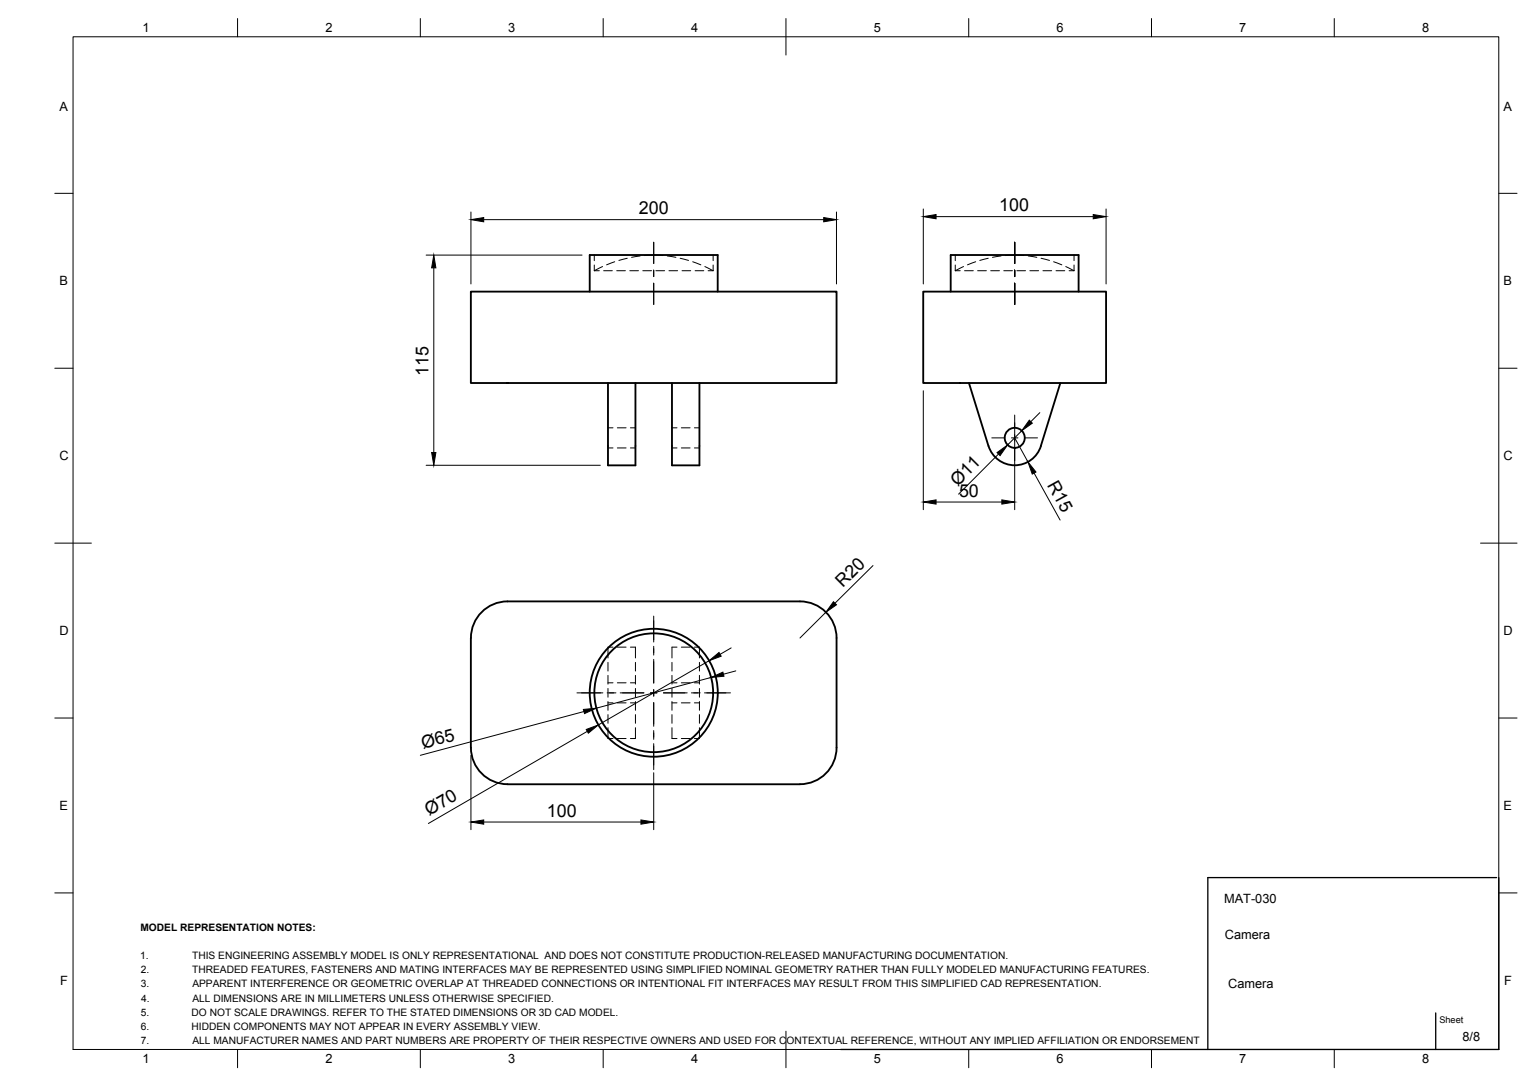
ISO-10303-21;
HEADER;
/* Generated by software containing ST-Developer
 * from STEP Tools, Inc. (www.steptools.com) 
 */

FILE_DESCRIPTION(
/* description */ ('STEP AP214'),
/* implementation_level */ '2;1');

FILE_NAME(
/* name */ 'Camera.step',
/* time_stamp */ '2026-11-14T06:43:04-08:00',
/* author */ (''),
/* organization */ (''),
/* preprocessor_version */ 'ST-DEVELOPER v20.2',
/* originating_system */ 'Autodesk Translation Framework v15.17.0.0',
/* authorisation */ '');

FILE_SCHEMA (('AUTOMOTIVE_DESIGN { 1 0 10303 214 3 1 1 }'));
ENDSEC;

DATA;
#10=MECHANICAL_DESIGN_GEOMETRIC_PRESENTATION_REPRESENTATION('',(#201),#5658);
#165=(
BOUNDED_SURFACE()
B_SPLINE_SURFACE(2,2,((#4850,#4851,#4852,#4853,#4854,#4855,#4856,#4857,
#4858),(#4859,#4860,#4861,#4862,#4863,#4864,#4865,#4866,#4867),(#4868,#4869,
#4870,#4871,#4872,#4873,#4874,#4875,#4876)),.UNSPECIFIED.,.F.,.T.,.F.)
B_SPLINE_SURFACE_WITH_KNOTS((3,3),(3,2,2,2,3),(-1.55552293509789,-1.0706447979528),
(-3.14159265358979,-1.5707963267949,0.,1.5707963267949,3.14159265358979),
 .UNSPECIFIED.)
GEOMETRIC_REPRESENTATION_ITEM()
RATIONAL_B_SPLINE_SURFACE(((1.,0.707106781186548,1.,0.707106781186548,1.,
0.707106781186548,1.,0.707106781186548,1.),(0.970755313150814,0.686427664801811,
0.970755313150814,0.686427664801811,0.970755313150814,0.686427664801811,
0.970755313150814,0.686427664801811,0.970755313150814),(1.,0.707106781186548,
1.,0.707106781186548,1.,0.707106781186548,1.,0.707106781186548,1.)))
REPRESENTATION_ITEM('')
SURFACE()
);
#179=SHAPE_REPRESENTATION_RELATIONSHIP('SRR','None',#5709,#190);
#190=ADVANCED_BREP_SHAPE_REPRESENTATION('',(#212),#5650);
#201=STYLED_ITEM('',(#5772),#212);
#212=MANIFOLD_SOLID_BREP('Body1',#3063);
#242=CYLINDRICAL_SURFACE('',#3279,5.5);
#243=CYLINDRICAL_SURFACE('',#3282,5.5);
#244=CYLINDRICAL_SURFACE('',#3285,35.);
#245=CYLINDRICAL_SURFACE('',#3290,32.5);
#246=CYLINDRICAL_SURFACE('',#3292,15.);
#247=CYLINDRICAL_SURFACE('',#3297,20.);
#248=CYLINDRICAL_SURFACE('',#3301,20.);
#249=CYLINDRICAL_SURFACE('',#3305,20.);
#250=CYLINDRICAL_SURFACE('',#3309,20.);
#251=CYLINDRICAL_SURFACE('',#3316,15.);
#299=FACE_BOUND('',#603,.T.);
#300=FACE_BOUND('',#604,.T.);
#301=FACE_BOUND('',#606,.T.);
#302=FACE_BOUND('',#608,.T.);
#303=FACE_BOUND('',#613,.T.);
#304=FACE_BOUND('',#615,.T.);
#305=FACE_BOUND('',#617,.T.);
#306=FACE_BOUND('',#619,.T.);
#376=FACE_OUTER_BOUND('',#586,.T.);
#377=FACE_OUTER_BOUND('',#587,.T.);
#378=FACE_OUTER_BOUND('',#588,.T.);
#379=FACE_OUTER_BOUND('',#589,.T.);
#380=FACE_OUTER_BOUND('',#590,.T.);
#381=FACE_OUTER_BOUND('',#591,.T.);
#382=FACE_OUTER_BOUND('',#592,.T.);
#383=FACE_OUTER_BOUND('',#593,.T.);
#384=FACE_OUTER_BOUND('',#594,.T.);
#385=FACE_OUTER_BOUND('',#595,.T.);
#386=FACE_OUTER_BOUND('',#596,.T.);
#387=FACE_OUTER_BOUND('',#597,.T.);
#388=FACE_OUTER_BOUND('',#598,.T.);
#389=FACE_OUTER_BOUND('',#599,.T.);
#390=FACE_OUTER_BOUND('',#600,.T.);
#391=FACE_OUTER_BOUND('',#601,.T.);
#392=FACE_OUTER_BOUND('',#602,.T.);
#393=FACE_OUTER_BOUND('',#605,.T.);
#394=FACE_OUTER_BOUND('',#607,.T.);
#395=FACE_OUTER_BOUND('',#609,.T.);
#396=FACE_OUTER_BOUND('',#610,.T.);
#397=FACE_OUTER_BOUND('',#611,.T.);
#398=FACE_OUTER_BOUND('',#612,.T.);
#399=FACE_OUTER_BOUND('',#614,.T.);
#400=FACE_OUTER_BOUND('',#616,.T.);
#401=FACE_OUTER_BOUND('',#618,.T.);
#586=EDGE_LOOP('',(#2158,#2159,#2160,#2161));
#587=EDGE_LOOP('',(#2162,#2163,#2164,#2165));
#588=EDGE_LOOP('',(#2166,#2167,#2168,#2169));
#589=EDGE_LOOP('',(#2170,#2171,#2172));
#590=EDGE_LOOP('',(#2173,#2174,#2175,#2176));
#591=EDGE_LOOP('',(#2177,#2178,#2179,#2180));
#592=EDGE_LOOP('',(#2181,#2182,#2183,#2184));
#593=EDGE_LOOP('',(#2185,#2186,#2187,#2188));
#594=EDGE_LOOP('',(#2189,#2190,#2191,#2192));
#595=EDGE_LOOP('',(#2193,#2194,#2195,#2196));
#596=EDGE_LOOP('',(#2197,#2198,#2199,#2200));
#597=EDGE_LOOP('',(#2201,#2202,#2203,#2204));
#598=EDGE_LOOP('',(#2205,#2206,#2207,#2208));
#599=EDGE_LOOP('',(#2209,#2210,#2211,#2212));
#600=EDGE_LOOP('',(#2213,#2214,#2215,#2216));
#601=EDGE_LOOP('',(#2217,#2218,#2219,#2220));
#602=EDGE_LOOP('',(#2221,#2222,#2223,#2224,#2225,#2226,#2227,#2228));
#603=EDGE_LOOP('',(#2229,#2230,#2231,#2232));
#604=EDGE_LOOP('',(#2233,#2234,#2235,#2236));
#605=EDGE_LOOP('',(#2237,#2238,#2239,#2240,#2241,#2242,#2243,#2244));
#606=EDGE_LOOP('',(#2245));
#607=EDGE_LOOP('',(#2246));
#608=EDGE_LOOP('',(#2247));
#609=EDGE_LOOP('',(#2248,#2249,#2250,#2251));
#610=EDGE_LOOP('',(#2252,#2253,#2254,#2255));
#611=EDGE_LOOP('',(#2256,#2257,#2258,#2259));
#612=EDGE_LOOP('',(#2260,#2261,#2262,#2263));
#613=EDGE_LOOP('',(#2264));
#614=EDGE_LOOP('',(#2265,#2266,#2267,#2268));
#615=EDGE_LOOP('',(#2269));
#616=EDGE_LOOP('',(#2270,#2271,#2272,#2273));
#617=EDGE_LOOP('',(#2274));
#618=EDGE_LOOP('',(#2275,#2276,#2277,#2278));
#619=EDGE_LOOP('',(#2279));
#810=LINE('',#4836,#1006);
#811=LINE('',#4842,#1007);
#812=LINE('',#4848,#1008);
#813=LINE('',#4884,#1009);
#814=LINE('',#4890,#1010);
#815=LINE('',#4893,#1011);
#816=LINE('',#4896,#1012);
#817=LINE('',#4898,#1013);
#818=LINE('',#4899,#1014);
#819=LINE('',#4902,#1015);
#820=LINE('',#4904,#1016);
#821=LINE('',#4905,#1017);
#822=LINE('',#4911,#1018);
#823=LINE('',#4914,#1019);
#824=LINE('',#4917,#1020);
#825=LINE('',#4919,#1021);
#826=LINE('',#4920,#1022);
#827=LINE('',#4925,#1023);
#828=LINE('',#4929,#1024);
#829=LINE('',#4931,#1025);
#830=LINE('',#4932,#1026);
#831=LINE('',#4937,#1027);
#832=LINE('',#4941,#1028);
#833=LINE('',#4943,#1029);
#834=LINE('',#4944,#1030);
#835=LINE('',#4949,#1031);
#836=LINE('',#4952,#1032);
#837=LINE('',#4953,#1033);
#838=LINE('',#4957,#1034);
#839=LINE('',#4959,#1035);
#840=LINE('',#4961,#1036);
#841=LINE('',#4962,#1037);
#842=LINE('',#4963,#1038);
#843=LINE('',#4964,#1039);
#844=LINE('',#4970,#1040);
#845=LINE('',#4974,#1041);
#846=LINE('',#4977,#1042);
#847=LINE('',#4978,#1043);
#848=LINE('',#4980,#1044);
#849=LINE('',#4981,#1045);
#1006=VECTOR('',#3778,5.5);
#1007=VECTOR('',#3785,5.5);
#1008=VECTOR('',#3792,35.);
#1009=VECTOR('',#3803,32.5);
#1010=VECTOR('',#3808,1000.);
#1011=VECTOR('',#3811,1000.);
#1012=VECTOR('',#3814,1000.);
#1013=VECTOR('',#3815,1000.);
#1014=VECTOR('',#3816,1000.);
#1015=VECTOR('',#3819,1000.);
#1016=VECTOR('',#3820,1000.);
#1017=VECTOR('',#3821,1000.);
#1018=VECTOR('',#3826,1000.);
#1019=VECTOR('',#3829,1000.);
#1020=VECTOR('',#3832,1000.);
#1021=VECTOR('',#3833,1000.);
#1022=VECTOR('',#3834,1000.);
#1023=VECTOR('',#3839,1000.);
#1024=VECTOR('',#3844,1000.);
#1025=VECTOR('',#3845,1000.);
#1026=VECTOR('',#3846,1000.);
#1027=VECTOR('',#3851,1000.);
#1028=VECTOR('',#3856,1000.);
#1029=VECTOR('',#3857,1000.);
#1030=VECTOR('',#3858,1000.);
#1031=VECTOR('',#3863,1000.);
#1032=VECTOR('',#3868,1000.);
#1033=VECTOR('',#3869,1000.);
#1034=VECTOR('',#3872,1000.);
#1035=VECTOR('',#3873,1000.);
#1036=VECTOR('',#3874,1000.);
#1037=VECTOR('',#3875,1000.);
#1038=VECTOR('',#3876,1000.);
#1039=VECTOR('',#3877,1000.);
#1040=VECTOR('',#3884,1000.);
#1041=VECTOR('',#3887,1000.);
#1042=VECTOR('',#3892,1000.);
#1043=VECTOR('',#3893,1000.);
#1044=VECTOR('',#3896,1000.);
#1045=VECTOR('',#3897,1000.);
#1201=CIRCLE('',#3280,5.5);
#1202=CIRCLE('',#3281,5.5);
#1203=CIRCLE('',#3283,5.5);
#1204=CIRCLE('',#3284,5.5);
#1205=CIRCLE('',#3286,35.);
#1206=CIRCLE('',#3287,35.);
#1207=CIRCLE('',#3288,32.5);
#1208=CIRCLE('',#3289,70.);
#1209=CIRCLE('',#3291,32.5);
#1210=CIRCLE('',#3293,15.);
#1211=CIRCLE('',#3294,15.);
#1212=CIRCLE('',#3298,20.);
#1213=CIRCLE('',#3299,20.);
#1214=CIRCLE('',#3302,20.);
#1215=CIRCLE('',#3303,20.);
#1216=CIRCLE('',#3306,20.);
#1217=CIRCLE('',#3307,20.);
#1218=CIRCLE('',#3310,20.);
#1219=CIRCLE('',#3311,20.);
#1220=CIRCLE('',#3317,15.);
#1221=CIRCLE('',#3318,15.);
#1374=VERTEX_POINT('',#4833);
#1375=VERTEX_POINT('',#4835);
#1376=VERTEX_POINT('',#4839);
#1377=VERTEX_POINT('',#4841);
#1378=VERTEX_POINT('',#4845);
#1379=VERTEX_POINT('',#4847);
#1380=VERTEX_POINT('',#4877);
#1381=VERTEX_POINT('',#4879);
#1382=VERTEX_POINT('',#4882);
#1383=VERTEX_POINT('',#4886);
#1384=VERTEX_POINT('',#4887);
#1385=VERTEX_POINT('',#4889);
#1386=VERTEX_POINT('',#4891);
#1387=VERTEX_POINT('',#4895);
#1388=VERTEX_POINT('',#4897);
#1389=VERTEX_POINT('',#4901);
#1390=VERTEX_POINT('',#4903);
#1391=VERTEX_POINT('',#4907);
#1392=VERTEX_POINT('',#4908);
#1393=VERTEX_POINT('',#4910);
#1394=VERTEX_POINT('',#4912);
#1395=VERTEX_POINT('',#4916);
#1396=VERTEX_POINT('',#4918);
#1397=VERTEX_POINT('',#4922);
#1398=VERTEX_POINT('',#4924);
#1399=VERTEX_POINT('',#4928);
#1400=VERTEX_POINT('',#4930);
#1401=VERTEX_POINT('',#4934);
#1402=VERTEX_POINT('',#4936);
#1403=VERTEX_POINT('',#4940);
#1404=VERTEX_POINT('',#4942);
#1405=VERTEX_POINT('',#4946);
#1406=VERTEX_POINT('',#4948);
#1407=VERTEX_POINT('',#4955);
#1408=VERTEX_POINT('',#4956);
#1409=VERTEX_POINT('',#4958);
#1410=VERTEX_POINT('',#4960);
#1411=VERTEX_POINT('',#4968);
#1412=VERTEX_POINT('',#4969);
#1413=VERTEX_POINT('',#4971);
#1414=VERTEX_POINT('',#4973);
#1662=EDGE_CURVE('',#1374,#1374,#1201,.T.);
#1663=EDGE_CURVE('',#1374,#1375,#810,.T.);
#1664=EDGE_CURVE('',#1375,#1375,#1202,.T.);
#1665=EDGE_CURVE('',#1376,#1376,#1203,.T.);
#1666=EDGE_CURVE('',#1376,#1377,#811,.T.);
#1667=EDGE_CURVE('',#1377,#1377,#1204,.T.);
#1668=EDGE_CURVE('',#1378,#1378,#1205,.T.);
#1669=EDGE_CURVE('',#1378,#1379,#812,.T.);
#1670=EDGE_CURVE('',#1379,#1379,#1206,.T.);
#1671=EDGE_CURVE('',#1380,#1380,#1207,.T.);
#1672=EDGE_CURVE('',#1380,#1381,#1208,.T.);
#1673=EDGE_CURVE('',#1382,#1382,#1209,.T.);
#1674=EDGE_CURVE('',#1382,#1380,#813,.T.);
#1675=EDGE_CURVE('',#1383,#1384,#1210,.T.);
#1676=EDGE_CURVE('',#1383,#1385,#814,.T.);
#1677=EDGE_CURVE('',#1385,#1386,#1211,.T.);
#1678=EDGE_CURVE('',#1384,#1386,#815,.T.);
#1679=EDGE_CURVE('',#1384,#1387,#816,.T.);
#1680=EDGE_CURVE('',#1386,#1388,#817,.T.);
#1681=EDGE_CURVE('',#1387,#1388,#818,.T.);
#1682=EDGE_CURVE('',#1389,#1383,#819,.T.);
#1683=EDGE_CURVE('',#1389,#1390,#820,.T.);
#1684=EDGE_CURVE('',#1390,#1385,#821,.T.);
#1685=EDGE_CURVE('',#1391,#1392,#1212,.T.);
#1686=EDGE_CURVE('',#1393,#1391,#822,.T.);
#1687=EDGE_CURVE('',#1393,#1394,#1213,.T.);
#1688=EDGE_CURVE('',#1394,#1392,#823,.T.);
#1689=EDGE_CURVE('',#1395,#1391,#824,.T.);
#1690=EDGE_CURVE('',#1396,#1395,#825,.T.);
#1691=EDGE_CURVE('',#1396,#1393,#826,.T.);
#1692=EDGE_CURVE('',#1397,#1395,#1214,.T.);
#1693=EDGE_CURVE('',#1398,#1397,#827,.T.);
#1694=EDGE_CURVE('',#1398,#1396,#1215,.T.);
#1695=EDGE_CURVE('',#1399,#1397,#828,.T.);
#1696=EDGE_CURVE('',#1400,#1399,#829,.T.);
#1697=EDGE_CURVE('',#1400,#1398,#830,.T.);
#1698=EDGE_CURVE('',#1401,#1399,#1216,.T.);
#1699=EDGE_CURVE('',#1402,#1401,#831,.T.);
#1700=EDGE_CURVE('',#1402,#1400,#1217,.T.);
#1701=EDGE_CURVE('',#1403,#1401,#832,.T.);
#1702=EDGE_CURVE('',#1404,#1403,#833,.T.);
#1703=EDGE_CURVE('',#1404,#1402,#834,.T.);
#1704=EDGE_CURVE('',#1405,#1403,#1218,.T.);
#1705=EDGE_CURVE('',#1406,#1405,#835,.T.);
#1706=EDGE_CURVE('',#1406,#1404,#1219,.T.);
#1707=EDGE_CURVE('',#1392,#1405,#836,.T.);
#1708=EDGE_CURVE('',#1394,#1406,#837,.T.);
#1709=EDGE_CURVE('',#1407,#1408,#838,.T.);
#1710=EDGE_CURVE('',#1408,#1409,#839,.T.);
#1711=EDGE_CURVE('',#1410,#1409,#840,.T.);
#1712=EDGE_CURVE('',#1407,#1410,#841,.T.);
#1713=EDGE_CURVE('',#1387,#1389,#842,.T.);
#1714=EDGE_CURVE('',#1388,#1390,#843,.T.);
#1715=EDGE_CURVE('',#1411,#1412,#844,.T.);
#1716=EDGE_CURVE('',#1412,#1413,#1220,.T.);
#1717=EDGE_CURVE('',#1414,#1413,#845,.T.);
#1718=EDGE_CURVE('',#1411,#1414,#1221,.T.);
#1719=EDGE_CURVE('',#1413,#1408,#846,.T.);
#1720=EDGE_CURVE('',#1414,#1407,#847,.T.);
#1721=EDGE_CURVE('',#1409,#1412,#848,.T.);
#1722=EDGE_CURVE('',#1410,#1411,#849,.T.);
#2158=ORIENTED_EDGE('',*,*,#1662,.F.);
#2159=ORIENTED_EDGE('',*,*,#1663,.T.);
#2160=ORIENTED_EDGE('',*,*,#1664,.T.);
#2161=ORIENTED_EDGE('',*,*,#1663,.F.);
#2162=ORIENTED_EDGE('',*,*,#1665,.F.);
#2163=ORIENTED_EDGE('',*,*,#1666,.T.);
#2164=ORIENTED_EDGE('',*,*,#1667,.T.);
#2165=ORIENTED_EDGE('',*,*,#1666,.F.);
#2166=ORIENTED_EDGE('',*,*,#1668,.F.);
#2167=ORIENTED_EDGE('',*,*,#1669,.T.);
#2168=ORIENTED_EDGE('',*,*,#1670,.T.);
#2169=ORIENTED_EDGE('',*,*,#1669,.F.);
#2170=ORIENTED_EDGE('',*,*,#1671,.F.);
#2171=ORIENTED_EDGE('',*,*,#1672,.T.);
#2172=ORIENTED_EDGE('',*,*,#1672,.F.);
#2173=ORIENTED_EDGE('',*,*,#1673,.F.);
#2174=ORIENTED_EDGE('',*,*,#1674,.T.);
#2175=ORIENTED_EDGE('',*,*,#1671,.T.);
#2176=ORIENTED_EDGE('',*,*,#1674,.F.);
#2177=ORIENTED_EDGE('',*,*,#1675,.F.);
#2178=ORIENTED_EDGE('',*,*,#1676,.T.);
#2179=ORIENTED_EDGE('',*,*,#1677,.T.);
#2180=ORIENTED_EDGE('',*,*,#1678,.F.);
#2181=ORIENTED_EDGE('',*,*,#1679,.F.);
#2182=ORIENTED_EDGE('',*,*,#1678,.T.);
#2183=ORIENTED_EDGE('',*,*,#1680,.T.);
#2184=ORIENTED_EDGE('',*,*,#1681,.F.);
#2185=ORIENTED_EDGE('',*,*,#1682,.F.);
#2186=ORIENTED_EDGE('',*,*,#1683,.T.);
#2187=ORIENTED_EDGE('',*,*,#1684,.T.);
#2188=ORIENTED_EDGE('',*,*,#1676,.F.);
#2189=ORIENTED_EDGE('',*,*,#1685,.F.);
#2190=ORIENTED_EDGE('',*,*,#1686,.F.);
#2191=ORIENTED_EDGE('',*,*,#1687,.T.);
#2192=ORIENTED_EDGE('',*,*,#1688,.T.);
#2193=ORIENTED_EDGE('',*,*,#1689,.F.);
#2194=ORIENTED_EDGE('',*,*,#1690,.F.);
#2195=ORIENTED_EDGE('',*,*,#1691,.T.);
#2196=ORIENTED_EDGE('',*,*,#1686,.T.);
#2197=ORIENTED_EDGE('',*,*,#1692,.F.);
#2198=ORIENTED_EDGE('',*,*,#1693,.F.);
#2199=ORIENTED_EDGE('',*,*,#1694,.T.);
#2200=ORIENTED_EDGE('',*,*,#1690,.T.);
#2201=ORIENTED_EDGE('',*,*,#1695,.F.);
#2202=ORIENTED_EDGE('',*,*,#1696,.F.);
#2203=ORIENTED_EDGE('',*,*,#1697,.T.);
#2204=ORIENTED_EDGE('',*,*,#1693,.T.);
#2205=ORIENTED_EDGE('',*,*,#1698,.F.);
#2206=ORIENTED_EDGE('',*,*,#1699,.F.);
#2207=ORIENTED_EDGE('',*,*,#1700,.T.);
#2208=ORIENTED_EDGE('',*,*,#1696,.T.);
#2209=ORIENTED_EDGE('',*,*,#1701,.F.);
#2210=ORIENTED_EDGE('',*,*,#1702,.F.);
#2211=ORIENTED_EDGE('',*,*,#1703,.T.);
#2212=ORIENTED_EDGE('',*,*,#1699,.T.);
#2213=ORIENTED_EDGE('',*,*,#1704,.F.);
#2214=ORIENTED_EDGE('',*,*,#1705,.F.);
#2215=ORIENTED_EDGE('',*,*,#1706,.T.);
#2216=ORIENTED_EDGE('',*,*,#1702,.T.);
#2217=ORIENTED_EDGE('',*,*,#1707,.F.);
#2218=ORIENTED_EDGE('',*,*,#1688,.F.);
#2219=ORIENTED_EDGE('',*,*,#1708,.T.);
#2220=ORIENTED_EDGE('',*,*,#1705,.T.);
#2221=ORIENTED_EDGE('',*,*,#1687,.F.);
#2222=ORIENTED_EDGE('',*,*,#1691,.F.);
#2223=ORIENTED_EDGE('',*,*,#1694,.F.);
#2224=ORIENTED_EDGE('',*,*,#1697,.F.);
#2225=ORIENTED_EDGE('',*,*,#1700,.F.);
#2226=ORIENTED_EDGE('',*,*,#1703,.F.);
#2227=ORIENTED_EDGE('',*,*,#1706,.F.);
#2228=ORIENTED_EDGE('',*,*,#1708,.F.);
#2229=ORIENTED_EDGE('',*,*,#1709,.T.);
#2230=ORIENTED_EDGE('',*,*,#1710,.T.);
#2231=ORIENTED_EDGE('',*,*,#1711,.F.);
#2232=ORIENTED_EDGE('',*,*,#1712,.F.);
#2233=ORIENTED_EDGE('',*,*,#1713,.F.);
#2234=ORIENTED_EDGE('',*,*,#1681,.T.);
#2235=ORIENTED_EDGE('',*,*,#1714,.T.);
#2236=ORIENTED_EDGE('',*,*,#1683,.F.);
#2237=ORIENTED_EDGE('',*,*,#1685,.T.);
#2238=ORIENTED_EDGE('',*,*,#1707,.T.);
#2239=ORIENTED_EDGE('',*,*,#1704,.T.);
#2240=ORIENTED_EDGE('',*,*,#1701,.T.);
#2241=ORIENTED_EDGE('',*,*,#1698,.T.);
#2242=ORIENTED_EDGE('',*,*,#1695,.T.);
#2243=ORIENTED_EDGE('',*,*,#1692,.T.);
#2244=ORIENTED_EDGE('',*,*,#1689,.T.);
#2245=ORIENTED_EDGE('',*,*,#1668,.T.);
#2246=ORIENTED_EDGE('',*,*,#1670,.F.);
#2247=ORIENTED_EDGE('',*,*,#1673,.T.);
#2248=ORIENTED_EDGE('',*,*,#1715,.T.);
#2249=ORIENTED_EDGE('',*,*,#1716,.T.);
#2250=ORIENTED_EDGE('',*,*,#1717,.F.);
#2251=ORIENTED_EDGE('',*,*,#1718,.F.);
#2252=ORIENTED_EDGE('',*,*,#1717,.T.);
#2253=ORIENTED_EDGE('',*,*,#1719,.T.);
#2254=ORIENTED_EDGE('',*,*,#1709,.F.);
#2255=ORIENTED_EDGE('',*,*,#1720,.F.);
#2256=ORIENTED_EDGE('',*,*,#1711,.T.);
#2257=ORIENTED_EDGE('',*,*,#1721,.T.);
#2258=ORIENTED_EDGE('',*,*,#1715,.F.);
#2259=ORIENTED_EDGE('',*,*,#1722,.F.);
#2260=ORIENTED_EDGE('',*,*,#1718,.T.);
#2261=ORIENTED_EDGE('',*,*,#1720,.T.);
#2262=ORIENTED_EDGE('',*,*,#1712,.T.);
#2263=ORIENTED_EDGE('',*,*,#1722,.T.);
#2264=ORIENTED_EDGE('',*,*,#1667,.F.);
#2265=ORIENTED_EDGE('',*,*,#1677,.F.);
#2266=ORIENTED_EDGE('',*,*,#1684,.F.);
#2267=ORIENTED_EDGE('',*,*,#1714,.F.);
#2268=ORIENTED_EDGE('',*,*,#1680,.F.);
#2269=ORIENTED_EDGE('',*,*,#1662,.T.);
#2270=ORIENTED_EDGE('',*,*,#1675,.T.);
#2271=ORIENTED_EDGE('',*,*,#1679,.T.);
#2272=ORIENTED_EDGE('',*,*,#1713,.T.);
#2273=ORIENTED_EDGE('',*,*,#1682,.T.);
#2274=ORIENTED_EDGE('',*,*,#1664,.F.);
#2275=ORIENTED_EDGE('',*,*,#1716,.F.);
#2276=ORIENTED_EDGE('',*,*,#1721,.F.);
#2277=ORIENTED_EDGE('',*,*,#1710,.F.);
#2278=ORIENTED_EDGE('',*,*,#1719,.F.);
#2279=ORIENTED_EDGE('',*,*,#1665,.T.);
#2801=PLANE('',#3295);
#2802=PLANE('',#3296);
#2803=PLANE('',#3300);
#2804=PLANE('',#3304);
#2805=PLANE('',#3308);
#2806=PLANE('',#3312);
#2807=PLANE('',#3313);
#2808=PLANE('',#3314);
#2809=PLANE('',#3315);
#2810=PLANE('',#3319);
#2811=PLANE('',#3320);
#2812=PLANE('',#3321);
#2813=PLANE('',#3322);
#2814=PLANE('',#3323);
#2815=PLANE('',#3324);
#2917=ADVANCED_FACE('',(#376),#242,.F.);
#2918=ADVANCED_FACE('',(#377),#243,.F.);
#2919=ADVANCED_FACE('',(#378),#244,.T.);
#2920=ADVANCED_FACE('',(#379),#165,.F.);
#2921=ADVANCED_FACE('',(#380),#245,.F.);
#2922=ADVANCED_FACE('',(#381),#246,.T.);
#2923=ADVANCED_FACE('',(#382),#2801,.F.);
#2924=ADVANCED_FACE('',(#383),#2802,.F.);
#2925=ADVANCED_FACE('',(#384),#247,.T.);
#2926=ADVANCED_FACE('',(#385),#2803,.T.);
#2927=ADVANCED_FACE('',(#386),#248,.T.);
#2928=ADVANCED_FACE('',(#387),#2804,.T.);
#2929=ADVANCED_FACE('',(#388),#249,.T.);
#2930=ADVANCED_FACE('',(#389),#2805,.T.);
#2931=ADVANCED_FACE('',(#390),#250,.T.);
#2932=ADVANCED_FACE('',(#391),#2806,.T.);
#2933=ADVANCED_FACE('',(#392,#299,#300),#2807,.T.);
#2934=ADVANCED_FACE('',(#393,#301),#2808,.F.);
#2935=ADVANCED_FACE('',(#394,#302),#2809,.F.);
#2936=ADVANCED_FACE('',(#395),#251,.T.);
#2937=ADVANCED_FACE('',(#396),#2810,.F.);
#2938=ADVANCED_FACE('',(#397),#2811,.F.);
#2939=ADVANCED_FACE('',(#398,#303),#2812,.T.);
#2940=ADVANCED_FACE('',(#399,#304),#2813,.F.);
#2941=ADVANCED_FACE('',(#400,#305),#2814,.T.);
#2942=ADVANCED_FACE('',(#401,#306),#2815,.F.);
#3063=CLOSED_SHELL('',(#2917,#2918,#2919,#2920,#2921,#2922,#2923,#2924,
#2925,#2926,#2927,#2928,#2929,#2930,#2931,#2932,#2933,#2934,#2935,#2936,
#2937,#2938,#2939,#2940,#2941,#2942));
#3278=AXIS2_PLACEMENT_3D('',#4831,#3772,#3773);
#3279=AXIS2_PLACEMENT_3D('',#4832,#3774,#3775);
#3280=AXIS2_PLACEMENT_3D('',#4834,#3776,#3777);
#3281=AXIS2_PLACEMENT_3D('',#4837,#3779,#3780);
#3282=AXIS2_PLACEMENT_3D('',#4838,#3781,#3782);
#3283=AXIS2_PLACEMENT_3D('',#4840,#3783,#3784);
#3284=AXIS2_PLACEMENT_3D('',#4843,#3786,#3787);
#3285=AXIS2_PLACEMENT_3D('',#4844,#3788,#3789);
#3286=AXIS2_PLACEMENT_3D('',#4846,#3790,#3791);
#3287=AXIS2_PLACEMENT_3D('',#4849,#3793,#3794);
#3288=AXIS2_PLACEMENT_3D('',#4878,#3795,#3796);
#3289=AXIS2_PLACEMENT_3D('',#4880,#3797,#3798);
#3290=AXIS2_PLACEMENT_3D('',#4881,#3799,#3800);
#3291=AXIS2_PLACEMENT_3D('',#4883,#3801,#3802);
#3292=AXIS2_PLACEMENT_3D('',#4885,#3804,#3805);
#3293=AXIS2_PLACEMENT_3D('',#4888,#3806,#3807);
#3294=AXIS2_PLACEMENT_3D('',#4892,#3809,#3810);
#3295=AXIS2_PLACEMENT_3D('',#4894,#3812,#3813);
#3296=AXIS2_PLACEMENT_3D('',#4900,#3817,#3818);
#3297=AXIS2_PLACEMENT_3D('',#4906,#3822,#3823);
#3298=AXIS2_PLACEMENT_3D('',#4909,#3824,#3825);
#3299=AXIS2_PLACEMENT_3D('',#4913,#3827,#3828);
#3300=AXIS2_PLACEMENT_3D('',#4915,#3830,#3831);
#3301=AXIS2_PLACEMENT_3D('',#4921,#3835,#3836);
#3302=AXIS2_PLACEMENT_3D('',#4923,#3837,#3838);
#3303=AXIS2_PLACEMENT_3D('',#4926,#3840,#3841);
#3304=AXIS2_PLACEMENT_3D('',#4927,#3842,#3843);
#3305=AXIS2_PLACEMENT_3D('',#4933,#3847,#3848);
#3306=AXIS2_PLACEMENT_3D('',#4935,#3849,#3850);
#3307=AXIS2_PLACEMENT_3D('',#4938,#3852,#3853);
#3308=AXIS2_PLACEMENT_3D('',#4939,#3854,#3855);
#3309=AXIS2_PLACEMENT_3D('',#4945,#3859,#3860);
#3310=AXIS2_PLACEMENT_3D('',#4947,#3861,#3862);
#3311=AXIS2_PLACEMENT_3D('',#4950,#3864,#3865);
#3312=AXIS2_PLACEMENT_3D('',#4951,#3866,#3867);
#3313=AXIS2_PLACEMENT_3D('',#4954,#3870,#3871);
#3314=AXIS2_PLACEMENT_3D('',#4965,#3878,#3879);
#3315=AXIS2_PLACEMENT_3D('',#4966,#3880,#3881);
#3316=AXIS2_PLACEMENT_3D('',#4967,#3882,#3883);
#3317=AXIS2_PLACEMENT_3D('',#4972,#3885,#3886);
#3318=AXIS2_PLACEMENT_3D('',#4975,#3888,#3889);
#3319=AXIS2_PLACEMENT_3D('',#4976,#3890,#3891);
#3320=AXIS2_PLACEMENT_3D('',#4979,#3894,#3895);
#3321=AXIS2_PLACEMENT_3D('',#4982,#3898,#3899);
#3322=AXIS2_PLACEMENT_3D('',#4983,#3900,#3901);
#3323=AXIS2_PLACEMENT_3D('',#4984,#3902,#3903);
#3324=AXIS2_PLACEMENT_3D('',#4985,#3904,#3905);
#3772=DIRECTION('axis',(0.,0.,1.));
#3773=DIRECTION('refdir',(1.,0.,0.));
#3774=DIRECTION('center_axis',(0.,1.,0.));
#3775=DIRECTION('ref_axis',(0.,0.,1.));
#3776=DIRECTION('center_axis',(0.,1.,0.));
#3777=DIRECTION('ref_axis',(0.,0.,1.));
#3778=DIRECTION('',(0.,1.,0.));
#3779=DIRECTION('center_axis',(0.,1.,0.));
#3780=DIRECTION('ref_axis',(0.,0.,1.));
#3781=DIRECTION('center_axis',(0.,1.,0.));
#3782=DIRECTION('ref_axis',(0.,0.,1.));
#3783=DIRECTION('center_axis',(0.,1.,0.));
#3784=DIRECTION('ref_axis',(0.,0.,1.));
#3785=DIRECTION('',(0.,1.,0.));
#3786=DIRECTION('center_axis',(0.,1.,0.));
#3787=DIRECTION('ref_axis',(0.,0.,1.));
#3788=DIRECTION('center_axis',(-1.,0.,-7.76407098792971E-16));
#3789=DIRECTION('ref_axis',(-7.76407098792971E-16,0.,1.));
#3790=DIRECTION('center_axis',(-1.,0.,-7.76407098792971E-16));
#3791=DIRECTION('ref_axis',(-7.76407098792971E-16,0.,1.));
#3792=DIRECTION('',(1.,0.,7.76407098792971E-16));
#3793=DIRECTION('center_axis',(-1.,0.,-7.76407098792971E-16));
#3794=DIRECTION('ref_axis',(-7.76407098792971E-16,0.,1.));
#3795=DIRECTION('center_axis',(-1.,0.,-7.76407098792971E-16));
#3796=DIRECTION('ref_axis',(-7.76407098792971E-16,0.,1.));
#3797=DIRECTION('center_axis',(-9.50824468372095E-32,-1.,1.22464679914735E-16));
#3798=DIRECTION('ref_axis',(7.73103237808434E-16,-1.22464679914735E-16,
-1.));
#3799=DIRECTION('center_axis',(-1.,0.,-7.76407098792971E-16));
#3800=DIRECTION('ref_axis',(-7.76407098792971E-16,0.,1.));
#3801=DIRECTION('center_axis',(-1.,0.,-7.76407098792971E-16));
#3802=DIRECTION('ref_axis',(-7.76407098792971E-16,0.,1.));
#3803=DIRECTION('',(-1.,0.,-7.76407098792971E-16));
#3804=DIRECTION('center_axis',(0.,-1.,0.));
#3805=DIRECTION('ref_axis',(0.,0.,-1.));
#3806=DIRECTION('center_axis',(0.,1.,0.));
#3807=DIRECTION('ref_axis',(0.,0.,1.));
#3808=DIRECTION('',(0.,-1.,0.));
#3809=DIRECTION('center_axis',(0.,1.,0.));
#3810=DIRECTION('ref_axis',(0.,0.,1.));
#3811=DIRECTION('',(0.,-1.,0.));
#3812=DIRECTION('center_axis',(0.295992012371146,0.,-0.955190414845375));
#3813=DIRECTION('ref_axis',(-0.955190414845375,0.,-0.295992012371146));
#3814=DIRECTION('',(0.955190414845375,0.,0.295992012371146));
#3815=DIRECTION('',(0.955190414845375,0.,0.295992012371146));
#3816=DIRECTION('',(0.,-1.,0.));
#3817=DIRECTION('center_axis',(0.295992012371146,0.,0.955190414845375));
#3818=DIRECTION('ref_axis',(0.955190414845375,0.,-0.295992012371146));
#3819=DIRECTION('',(-0.955190414845375,0.,0.295992012371146));
#3820=DIRECTION('',(0.,-1.,0.));
#3821=DIRECTION('',(-0.955190414845375,0.,0.295992012371146));
#3822=DIRECTION('center_axis',(1.,0.,0.));
#3823=DIRECTION('ref_axis',(0.,0.,-1.));
#3824=DIRECTION('center_axis',(1.,0.,0.));
#3825=DIRECTION('ref_axis',(0.,0.,1.));
#3826=DIRECTION('',(1.,0.,0.));
#3827=DIRECTION('center_axis',(1.,0.,0.));
#3828=DIRECTION('ref_axis',(0.,0.,1.));
#3829=DIRECTION('',(1.,0.,0.));
#3830=DIRECTION('center_axis',(0.,-1.,0.));
#3831=DIRECTION('ref_axis',(0.,0.,-1.));
#3832=DIRECTION('',(0.,0.,-1.));
#3833=DIRECTION('',(1.,0.,0.));
#3834=DIRECTION('',(0.,0.,-1.));
#3835=DIRECTION('center_axis',(1.,0.,0.));
#3836=DIRECTION('ref_axis',(0.,0.,-1.));
#3837=DIRECTION('center_axis',(1.,0.,0.));
#3838=DIRECTION('ref_axis',(0.,0.,1.));
#3839=DIRECTION('',(1.,0.,0.));
#3840=DIRECTION('center_axis',(1.,0.,0.));
#3841=DIRECTION('ref_axis',(0.,0.,1.));
#3842=DIRECTION('center_axis',(0.,8.67361737988404E-17,1.));
#3843=DIRECTION('ref_axis',(0.,-1.,8.67361737988404E-17));
#3844=DIRECTION('',(0.,-1.,8.67361737988404E-17));
#3845=DIRECTION('',(1.,0.,0.));
#3846=DIRECTION('',(0.,-1.,8.67361737988404E-17));
#3847=DIRECTION('center_axis',(1.,0.,0.));
#3848=DIRECTION('ref_axis',(0.,0.,-1.));
#3849=DIRECTION('center_axis',(1.,0.,0.));
#3850=DIRECTION('ref_axis',(0.,0.,1.));
#3851=DIRECTION('',(1.,0.,0.));
#3852=DIRECTION('center_axis',(1.,0.,0.));
#3853=DIRECTION('ref_axis',(0.,0.,1.));
#3854=DIRECTION('center_axis',(0.,1.,0.));
#3855=DIRECTION('ref_axis',(0.,0.,1.));
#3856=DIRECTION('',(0.,0.,1.));
#3857=DIRECTION('',(1.,0.,0.));
#3858=DIRECTION('',(0.,0.,1.));
#3859=DIRECTION('center_axis',(1.,0.,0.));
#3860=DIRECTION('ref_axis',(0.,0.,-1.));
#3861=DIRECTION('center_axis',(1.,0.,0.));
#3862=DIRECTION('ref_axis',(0.,0.,-1.));
#3863=DIRECTION('',(1.,0.,0.));
#3864=DIRECTION('center_axis',(1.,0.,0.));
#3865=DIRECTION('ref_axis',(0.,0.,-1.));
#3866=DIRECTION('center_axis',(0.,-8.67361737988404E-17,-1.));
#3867=DIRECTION('ref_axis',(0.,1.,-8.67361737988404E-17));
#3868=DIRECTION('',(0.,1.,-8.67361737988404E-17));
#3869=DIRECTION('',(0.,1.,-8.67361737988404E-17));
#3870=DIRECTION('center_axis',(-1.,0.,0.));
#3871=DIRECTION('ref_axis',(0.,0.,1.));
#3872=DIRECTION('',(0.,-1.,0.));
#3873=DIRECTION('',(0.,0.,-1.));
#3874=DIRECTION('',(0.,-1.,0.));
#3875=DIRECTION('',(0.,0.,-1.));
#3876=DIRECTION('',(0.,0.,-1.));
#3877=DIRECTION('',(0.,0.,-1.));
#3878=DIRECTION('center_axis',(-1.,0.,0.));
#3879=DIRECTION('ref_axis',(0.,0.,1.));
#3880=DIRECTION('center_axis',(-1.,0.,-7.76407098792971E-16));
#3881=DIRECTION('ref_axis',(-7.76407098792971E-16,0.,1.));
#3882=DIRECTION('center_axis',(0.,-1.,0.));
#3883=DIRECTION('ref_axis',(0.,0.,-1.));
#3884=DIRECTION('',(0.,-1.,0.));
#3885=DIRECTION('center_axis',(0.,1.,0.));
#3886=DIRECTION('ref_axis',(0.,0.,1.));
#3887=DIRECTION('',(0.,-1.,0.));
#3888=DIRECTION('center_axis',(0.,1.,0.));
#3889=DIRECTION('ref_axis',(0.,0.,1.));
#3890=DIRECTION('center_axis',(0.295992012371146,0.,-0.955190414845375));
#3891=DIRECTION('ref_axis',(-0.955190414845375,0.,-0.295992012371146));
#3892=DIRECTION('',(0.955190414845375,0.,0.295992012371146));
#3893=DIRECTION('',(0.955190414845375,0.,0.295992012371146));
#3894=DIRECTION('center_axis',(0.295992012371146,0.,0.955190414845375));
#3895=DIRECTION('ref_axis',(0.955190414845375,0.,-0.295992012371146));
#3896=DIRECTION('',(-0.955190414845375,0.,0.295992012371146));
#3897=DIRECTION('',(-0.955190414845375,0.,0.295992012371146));
#3898=DIRECTION('center_axis',(0.,1.,0.));
#3899=DIRECTION('ref_axis',(0.,0.,1.));
#3900=DIRECTION('center_axis',(0.,1.,0.));
#3901=DIRECTION('ref_axis',(0.,0.,1.));
#3902=DIRECTION('center_axis',(0.,1.,0.));
#3903=DIRECTION('ref_axis',(0.,0.,1.));
#3904=DIRECTION('center_axis',(0.,1.,0.));
#3905=DIRECTION('ref_axis',(0.,0.,1.));
#4831=CARTESIAN_POINT('',(0.,0.,0.));
#4832=CARTESIAN_POINT('Origin',(-80.,-100.,-1.54074395550979E-30));
#4833=CARTESIAN_POINT('',(-80.,-25.,-5.5));
#4834=CARTESIAN_POINT('Origin',(-80.,-25.,-1.54074395550979E-30));
#4835=CARTESIAN_POINT('',(-80.,-10.,-5.5));
#4836=CARTESIAN_POINT('',(-80.,-100.,-5.5));
#4837=CARTESIAN_POINT('Origin',(-80.,-10.,-1.54074395550979E-30));
#4838=CARTESIAN_POINT('Origin',(-80.,-100.,-1.54074395550979E-30));
#4839=CARTESIAN_POINT('',(-80.,10.,-5.5));
#4840=CARTESIAN_POINT('Origin',(-80.,10.,-1.54074395550979E-30));
#4841=CARTESIAN_POINT('',(-80.,25.,-5.5));
#4842=CARTESIAN_POINT('',(-80.,-100.,-5.5));
#4843=CARTESIAN_POINT('Origin',(-80.,25.,-1.54074395550979E-30));
#4844=CARTESIAN_POINT('Origin',(20.,0.,-6.12323399573677E-15));
#4845=CARTESIAN_POINT('',(7.54951656745106E-14,-4.28626379701574E-15,-35.));
#4846=CARTESIAN_POINT('Origin',(4.85722573273506E-14,0.,-2.16513759715961E-14));
#4847=CARTESIAN_POINT('',(20.0000000000001,-4.28626379701574E-15,-35.));
#4848=CARTESIAN_POINT('',(20.,-4.28626379701574E-15,-35.));
#4849=CARTESIAN_POINT('Origin',(20.,0.,-6.12323399573675E-15));
#4850=CARTESIAN_POINT('Ctrl Pts',(20.,0.,-2.32063937709169E-15));
#4851=CARTESIAN_POINT('Ctrl Pts',(20.,3.83568392226736E-15,-2.32063937709169E-15));
#4852=CARTESIAN_POINT('Ctrl Pts',(20.,3.83568392226736E-15,-6.15632329935905E-15));
#4853=CARTESIAN_POINT('Ctrl Pts',(20.,3.83568392226736E-15,-9.99200722162641E-15));
#4854=CARTESIAN_POINT('Ctrl Pts',(20.,0.,-9.99200722162641E-15));
#4855=CARTESIAN_POINT('Ctrl Pts',(20.,-3.83568392226736E-15,-9.99200722162641E-15));
#4856=CARTESIAN_POINT('Ctrl Pts',(20.,-3.83568392226736E-15,-6.15632329935905E-15));
#4857=CARTESIAN_POINT('Ctrl Pts',(20.,-3.83568392226736E-15,-2.32063937709169E-15));
#4858=CARTESIAN_POINT('Ctrl Pts',(20.,0.,-2.32063937709169E-15));
#4859=CARTESIAN_POINT('Ctrl Pts',(19.735608974744,0.,-17.3092179814268));
#4860=CARTESIAN_POINT('Ctrl Pts',(19.735608974744,-17.3092179814268,-17.3092179814268));
#4861=CARTESIAN_POINT('Ctrl Pts',(19.7356089747439,-17.3092179814268,-6.36159836822499E-15));
#4862=CARTESIAN_POINT('Ctrl Pts',(19.7356089747439,-17.3092179814268,17.3092179814268));
#4863=CARTESIAN_POINT('Ctrl Pts',(19.7356089747439,0.,17.3092179814268));
#4864=CARTESIAN_POINT('Ctrl Pts',(19.7356089747439,17.3092179814268,17.3092179814268));
#4865=CARTESIAN_POINT('Ctrl Pts',(19.7356089747439,17.3092179814268,-6.36159836822499E-15));
#4866=CARTESIAN_POINT('Ctrl Pts',(19.735608974744,17.3092179814268,-17.3092179814268));
#4867=CARTESIAN_POINT('Ctrl Pts',(19.735608974744,0.,-17.3092179814268));
#4868=CARTESIAN_POINT('Ctrl Pts',(11.433857869888,0.,-32.5));
#4869=CARTESIAN_POINT('Ctrl Pts',(11.433857869888,-32.5,-32.5));
#4870=CARTESIAN_POINT('Ctrl Pts',(11.433857869888,-32.5,-1.28071368584476E-14));
#4871=CARTESIAN_POINT('Ctrl Pts',(11.4338578698879,-32.5,32.5));
#4872=CARTESIAN_POINT('Ctrl Pts',(11.4338578698879,0.,32.5));
#4873=CARTESIAN_POINT('Ctrl Pts',(11.4338578698879,32.5,32.5));
#4874=CARTESIAN_POINT('Ctrl Pts',(11.433857869888,32.5,-1.28071368584476E-14));
#4875=CARTESIAN_POINT('Ctrl Pts',(11.433857869888,32.5,-32.5));
#4876=CARTESIAN_POINT('Ctrl Pts',(11.433857869888,0.,-32.5));
#4877=CARTESIAN_POINT('',(11.433857869888,3.9801020972289E-15,-32.5));
#4878=CARTESIAN_POINT('Origin',(11.433857869888,0.,-1.27740475548253E-14));
#4879=CARTESIAN_POINT('',(20.,0.,-6.12323399573677E-15));
#4880=CARTESIAN_POINT('Origin',(-49.9918354814302,1.30926481293404E-16,
1.06909585183706));
#4881=CARTESIAN_POINT('Origin',(20.,0.,-6.12323399573677E-15));
#4882=CARTESIAN_POINT('',(20.0000000000001,-3.9801020972289E-15,-32.5));
#4883=CARTESIAN_POINT('Origin',(20.,0.,-6.12323399573675E-15));
#4884=CARTESIAN_POINT('',(20.,-3.9801020972289E-15,-32.5));
#4885=CARTESIAN_POINT('Origin',(-80.,25.,-1.54074395550979E-30));
#4886=CARTESIAN_POINT('',(-84.4398801855672,-10.,-14.3278562226806));
#4887=CARTESIAN_POINT('',(-84.4398801855672,-10.,14.3278562226806));
#4888=CARTESIAN_POINT('Origin',(-80.,-10.,-1.54074395550979E-30));
#4889=CARTESIAN_POINT('',(-84.4398801855672,-25.,-14.3278562226806));
#4890=CARTESIAN_POINT('',(-84.4398801855672,25.,-14.3278562226806));
#4891=CARTESIAN_POINT('',(-84.4398801855672,-25.,14.3278562226806));
#4892=CARTESIAN_POINT('Origin',(-80.,-25.,-1.54074395550979E-30));
#4893=CARTESIAN_POINT('',(-84.4398801855672,25.,14.3278562226806));
#4894=CARTESIAN_POINT('Origin',(-84.4398801855672,25.,14.3278562226806));
#4895=CARTESIAN_POINT('',(-50.,-10.,25.));
#4896=CARTESIAN_POINT('',(-84.4398801855672,-10.,14.3278562226806));
#4897=CARTESIAN_POINT('',(-50.,-25.,25.));
#4898=CARTESIAN_POINT('',(-84.4398801855672,-25.,14.3278562226806));
#4899=CARTESIAN_POINT('',(-50.,25.,25.));
#4900=CARTESIAN_POINT('Origin',(-50.,25.,-25.));
#4901=CARTESIAN_POINT('',(-50.,-10.,-25.));
#4902=CARTESIAN_POINT('',(-50.,-10.,-25.));
#4903=CARTESIAN_POINT('',(-50.,-25.,-25.));
#4904=CARTESIAN_POINT('',(-50.,25.,-25.));
#4905=CARTESIAN_POINT('',(-50.,-25.,-25.));
#4906=CARTESIAN_POINT('Origin',(-50.,-80.,-30.));
#4907=CARTESIAN_POINT('',(0.,-100.,-30.));
#4908=CARTESIAN_POINT('',(0.,-80.,-50.));
#4909=CARTESIAN_POINT('Origin',(0.,-80.,-30.));
#4910=CARTESIAN_POINT('',(-50.,-100.,-30.));
#4911=CARTESIAN_POINT('',(-50.,-100.,-30.));
#4912=CARTESIAN_POINT('',(-50.,-80.,-50.));
#4913=CARTESIAN_POINT('Origin',(-50.,-80.,-30.));
#4914=CARTESIAN_POINT('',(-50.,-80.,-50.));
#4915=CARTESIAN_POINT('Origin',(-50.,-100.,-30.));
#4916=CARTESIAN_POINT('',(0.,-100.,30.));
#4917=CARTESIAN_POINT('',(0.,-100.,-30.));
#4918=CARTESIAN_POINT('',(-50.,-100.,30.));
#4919=CARTESIAN_POINT('',(-50.,-100.,30.));
#4920=CARTESIAN_POINT('',(-50.,-100.,-30.));
#4921=CARTESIAN_POINT('Origin',(-50.,-80.,30.));
#4922=CARTESIAN_POINT('',(0.,-80.,50.));
#4923=CARTESIAN_POINT('Origin',(0.,-80.,30.));
#4924=CARTESIAN_POINT('',(-50.,-80.,50.));
#4925=CARTESIAN_POINT('',(-50.,-80.,50.));
#4926=CARTESIAN_POINT('Origin',(-50.,-80.,30.));
#4927=CARTESIAN_POINT('Origin',(-50.,-80.,50.));
#4928=CARTESIAN_POINT('',(0.,80.,50.));
#4929=CARTESIAN_POINT('',(0.,-80.,50.));
#4930=CARTESIAN_POINT('',(-50.,80.,50.));
#4931=CARTESIAN_POINT('',(-50.,80.,50.));
#4932=CARTESIAN_POINT('',(-50.,-80.,50.));
#4933=CARTESIAN_POINT('Origin',(-50.,80.,30.));
#4934=CARTESIAN_POINT('',(0.,100.,30.));
#4935=CARTESIAN_POINT('Origin',(0.,80.,30.));
#4936=CARTESIAN_POINT('',(-50.,100.,30.));
#4937=CARTESIAN_POINT('',(-50.,100.,30.));
#4938=CARTESIAN_POINT('Origin',(-50.,80.,30.));
#4939=CARTESIAN_POINT('Origin',(-50.,100.,-30.));
#4940=CARTESIAN_POINT('',(0.,100.,-30.));
#4941=CARTESIAN_POINT('',(0.,100.,-30.));
#4942=CARTESIAN_POINT('',(-50.,100.,-30.));
#4943=CARTESIAN_POINT('',(-50.,100.,-30.));
#4944=CARTESIAN_POINT('',(-50.,100.,-30.));
#4945=CARTESIAN_POINT('Origin',(-50.,80.,-30.));
#4946=CARTESIAN_POINT('',(0.,80.,-50.));
#4947=CARTESIAN_POINT('Origin',(0.,80.,-30.));
#4948=CARTESIAN_POINT('',(-50.,80.,-50.));
#4949=CARTESIAN_POINT('',(-50.,80.,-50.));
#4950=CARTESIAN_POINT('Origin',(-50.,80.,-30.));
#4951=CARTESIAN_POINT('Origin',(-50.,-80.,-50.));
#4952=CARTESIAN_POINT('',(0.,-80.,-50.));
#4953=CARTESIAN_POINT('',(-50.,-80.,-50.));
#4954=CARTESIAN_POINT('Origin',(-50.,-80.,-30.));
#4955=CARTESIAN_POINT('',(-50.,25.,25.));
#4956=CARTESIAN_POINT('',(-50.,10.,25.));
#4957=CARTESIAN_POINT('',(-50.,25.,25.));
#4958=CARTESIAN_POINT('',(-50.,10.,-25.));
#4959=CARTESIAN_POINT('',(-50.,10.,25.));
#4960=CARTESIAN_POINT('',(-50.,25.,-25.));
#4961=CARTESIAN_POINT('',(-50.,25.,-25.));
#4962=CARTESIAN_POINT('',(-50.,25.,25.));
#4963=CARTESIAN_POINT('',(-50.,-10.,25.));
#4964=CARTESIAN_POINT('',(-50.,-25.,25.));
#4965=CARTESIAN_POINT('Origin',(0.,-80.,-30.));
#4966=CARTESIAN_POINT('Origin',(20.,0.,2.0344769428144E-29));
#4967=CARTESIAN_POINT('Origin',(-80.,25.,-1.54074395550979E-30));
#4968=CARTESIAN_POINT('',(-84.4398801855672,25.,-14.3278562226806));
#4969=CARTESIAN_POINT('',(-84.4398801855672,10.,-14.3278562226806));
#4970=CARTESIAN_POINT('',(-84.4398801855672,25.,-14.3278562226806));
#4971=CARTESIAN_POINT('',(-84.4398801855672,10.,14.3278562226806));
#4972=CARTESIAN_POINT('Origin',(-80.,10.,-1.54074395550979E-30));
#4973=CARTESIAN_POINT('',(-84.4398801855672,25.,14.3278562226806));
#4974=CARTESIAN_POINT('',(-84.4398801855672,25.,14.3278562226806));
#4975=CARTESIAN_POINT('Origin',(-80.,25.,-1.54074395550979E-30));
#4976=CARTESIAN_POINT('Origin',(-84.4398801855672,25.,14.3278562226806));
#4977=CARTESIAN_POINT('',(-84.4398801855672,10.,14.3278562226806));
#4978=CARTESIAN_POINT('',(-84.4398801855672,25.,14.3278562226806));
#4979=CARTESIAN_POINT('Origin',(-50.,25.,-25.));
#4980=CARTESIAN_POINT('',(-50.,10.,-25.));
#4981=CARTESIAN_POINT('',(-50.,25.,-25.));
#4982=CARTESIAN_POINT('Origin',(-80.,25.,-1.54074395550979E-30));
#4983=CARTESIAN_POINT('Origin',(-80.,-25.,-1.54074395550979E-30));
#4984=CARTESIAN_POINT('Origin',(-80.,-10.,-1.54074395550979E-30));
#4985=CARTESIAN_POINT('Origin',(-80.,10.,-1.54074395550979E-30));
#5637=UNCERTAINTY_MEASURE_WITH_UNIT(LENGTH_MEASURE(0.01),#5659,
'DISTANCE_ACCURACY_VALUE',
'Maximum model space distance between geometric entities at asserted c
onnectivities');
#5645=UNCERTAINTY_MEASURE_WITH_UNIT(LENGTH_MEASURE(0.01),#5659,
'DISTANCE_ACCURACY_VALUE',
'Maximum model space distance between geometric entities at asserted c
onnectivities');
#5650=(
GEOMETRIC_REPRESENTATION_CONTEXT(3)
GLOBAL_UNCERTAINTY_ASSIGNED_CONTEXT((#5637))
GLOBAL_UNIT_ASSIGNED_CONTEXT((#5659,#5661,#5662))
REPRESENTATION_CONTEXT('','3D')
);
#5658=(
GEOMETRIC_REPRESENTATION_CONTEXT(3)
GLOBAL_UNCERTAINTY_ASSIGNED_CONTEXT((#5645))
GLOBAL_UNIT_ASSIGNED_CONTEXT((#5659,#5661,#5662))
REPRESENTATION_CONTEXT('','3D')
);
#5659=(
LENGTH_UNIT()
NAMED_UNIT(*)
SI_UNIT(.MILLI.,.METRE.)
);
#5661=(
NAMED_UNIT(*)
PLANE_ANGLE_UNIT()
SI_UNIT($,.RADIAN.)
);
#5662=(
NAMED_UNIT(*)
SI_UNIT($,.STERADIAN.)
SOLID_ANGLE_UNIT()
);
#5667=SHAPE_DEFINITION_REPRESENTATION(#5679,#5709);
#5679=PRODUCT_DEFINITION_SHAPE('',$,#5722);
#5709=SHAPE_REPRESENTATION('',(#3278),#5650);
#5717=PRODUCT_DEFINITION_CONTEXT('part definition',#5755,'design');
#5722=PRODUCT_DEFINITION('Camera','Camera',#5734,#5717);
#5734=PRODUCT_DEFINITION_FORMATION('',$,#5761);
#5755=APPLICATION_CONTEXT(
'Core Data for Automotive Mechanical Design Process');
#5756=PRODUCT_CONTEXT('part definition',#5755,'mechanical');
#5761=PRODUCT('Camera','Camera',$,(#5756));
#5772=PRESENTATION_STYLE_ASSIGNMENT((#5777));
#5777=SURFACE_STYLE_USAGE(.BOTH.,#5782);
#5782=SURFACE_SIDE_STYLE('',(#5787));
#5787=SURFACE_STYLE_FILL_AREA(#5792);
#5792=FILL_AREA_STYLE('Opaque(227,224,212)',(#5797));
#5797=FILL_AREA_STYLE_COLOUR('Opaque(227,224,212)',#5802);
#5802=COLOUR_RGB('Opaque(227,224,212)',0.890196078431372,0.87843137254902,
0.831372549019608);
ENDSEC;
END-ISO-10303-21;
